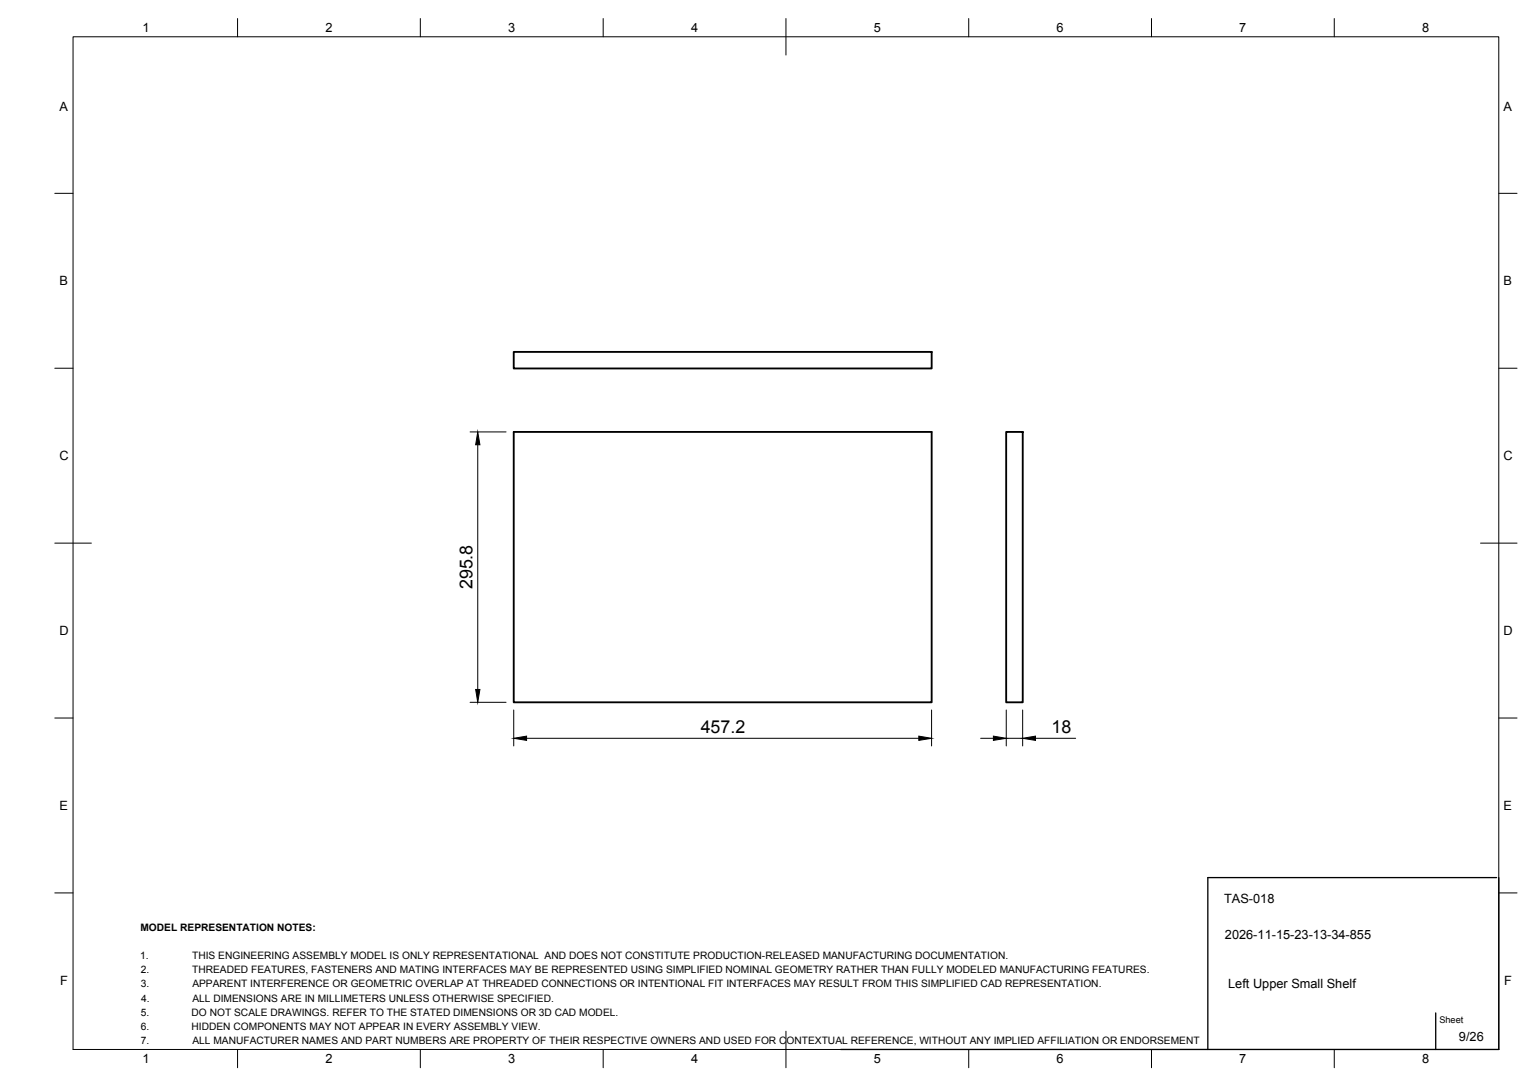
ISO-10303-21;
HEADER;
/* Generated by software containing ST-Developer
 * from STEP Tools, Inc. (www.steptools.com) 
 */

FILE_DESCRIPTION(
/* description */ (''),
/* implementation_level */ '2;1');

FILE_NAME(
/* name */ 'Left Upper Small Shelf.step',
/* time_stamp */ '2026-11-15T15:17:57-08:00',
/* author */ (''),
/* organization */ (''),
/* preprocessor_version */ 'ST-DEVELOPER v20.2',
/* originating_system */ 'Autodesk Translation Framework v15.17.0.0',
/* authorisation */ '');

FILE_SCHEMA (('AUTOMOTIVE_DESIGN { 1 0 10303 214 3 1 1 }'));
ENDSEC;

DATA;
#10=MECHANICAL_DESIGN_GEOMETRIC_PRESENTATION_REPRESENTATION('',(#184),#3723);
#136=SHAPE_REPRESENTATION_RELATIONSHIP('SRR','None',#3817,#160);
#160=ADVANCED_BREP_SHAPE_REPRESENTATION('',(#208),#3706);
#184=STYLED_ITEM('',(#3944),#208);
#208=MANIFOLD_SOLID_BREP('Body1',#2032);
#264=FACE_OUTER_BOUND('',#390,.T.);
#265=FACE_OUTER_BOUND('',#391,.T.);
#266=FACE_OUTER_BOUND('',#392,.T.);
#267=FACE_OUTER_BOUND('',#393,.T.);
#268=FACE_OUTER_BOUND('',#394,.T.);
#269=FACE_OUTER_BOUND('',#395,.T.);
#390=EDGE_LOOP('',(#1461,#1462,#1463,#1464));
#391=EDGE_LOOP('',(#1465,#1466,#1467,#1468));
#392=EDGE_LOOP('',(#1469,#1470,#1471,#1472));
#393=EDGE_LOOP('',(#1473,#1474,#1475,#1476));
#394=EDGE_LOOP('',(#1477,#1478,#1479,#1480));
#395=EDGE_LOOP('',(#1481,#1482,#1483,#1484));
#550=LINE('',#3281,#772);
#551=LINE('',#3283,#773);
#552=LINE('',#3285,#774);
#553=LINE('',#3286,#775);
#554=LINE('',#3289,#776);
#555=LINE('',#3291,#777);
#556=LINE('',#3292,#778);
#557=LINE('',#3295,#779);
#558=LINE('',#3297,#780);
#559=LINE('',#3298,#781);
#560=LINE('',#3300,#782);
#561=LINE('',#3301,#783);
#772=VECTOR('',#2682,0.708661417322828);
#773=VECTOR('',#2683,18.);
#774=VECTOR('',#2684,0.708661417322828);
#775=VECTOR('',#2685,18.);
#776=VECTOR('',#2688,11.6456692913386);
#777=VECTOR('',#2689,11.6456692913386);
#778=VECTOR('',#2690,18.);
#779=VECTOR('',#2693,0.708661417322839);
#780=VECTOR('',#2694,0.708661417322839);
#781=VECTOR('',#2695,18.);
#782=VECTOR('',#2698,11.6456692913386);
#783=VECTOR('',#2699,11.6456692913386);
#971=VERTEX_POINT('',#3279);
#972=VERTEX_POINT('',#3280);
#973=VERTEX_POINT('',#3282);
#974=VERTEX_POINT('',#3284);
#975=VERTEX_POINT('',#3288);
#976=VERTEX_POINT('',#3290);
#977=VERTEX_POINT('',#3294);
#978=VERTEX_POINT('',#3296);
#1152=EDGE_CURVE('',#971,#972,#550,.T.);
#1153=EDGE_CURVE('',#971,#973,#551,.T.);
#1154=EDGE_CURVE('',#973,#974,#552,.T.);
#1155=EDGE_CURVE('',#972,#974,#553,.T.);
#1156=EDGE_CURVE('',#972,#975,#554,.T.);
#1157=EDGE_CURVE('',#974,#976,#555,.T.);
#1158=EDGE_CURVE('',#975,#976,#556,.T.);
#1159=EDGE_CURVE('',#975,#977,#557,.T.);
#1160=EDGE_CURVE('',#976,#978,#558,.T.);
#1161=EDGE_CURVE('',#977,#978,#559,.T.);
#1162=EDGE_CURVE('',#977,#971,#560,.T.);
#1163=EDGE_CURVE('',#978,#973,#561,.T.);
#1461=ORIENTED_EDGE('',*,*,#1152,.F.);
#1462=ORIENTED_EDGE('',*,*,#1153,.T.);
#1463=ORIENTED_EDGE('',*,*,#1154,.T.);
#1464=ORIENTED_EDGE('',*,*,#1155,.F.);
#1465=ORIENTED_EDGE('',*,*,#1156,.F.);
#1466=ORIENTED_EDGE('',*,*,#1155,.T.);
#1467=ORIENTED_EDGE('',*,*,#1157,.T.);
#1468=ORIENTED_EDGE('',*,*,#1158,.F.);
#1469=ORIENTED_EDGE('',*,*,#1159,.F.);
#1470=ORIENTED_EDGE('',*,*,#1158,.T.);
#1471=ORIENTED_EDGE('',*,*,#1160,.T.);
#1472=ORIENTED_EDGE('',*,*,#1161,.F.);
#1473=ORIENTED_EDGE('',*,*,#1162,.F.);
#1474=ORIENTED_EDGE('',*,*,#1161,.T.);
#1475=ORIENTED_EDGE('',*,*,#1163,.T.);
#1476=ORIENTED_EDGE('',*,*,#1153,.F.);
#1477=ORIENTED_EDGE('',*,*,#1154,.F.);
#1478=ORIENTED_EDGE('',*,*,#1163,.F.);
#1479=ORIENTED_EDGE('',*,*,#1160,.F.);
#1480=ORIENTED_EDGE('',*,*,#1157,.F.);
#1481=ORIENTED_EDGE('',*,*,#1162,.T.);
#1482=ORIENTED_EDGE('',*,*,#1152,.T.);
#1483=ORIENTED_EDGE('',*,*,#1156,.T.);
#1484=ORIENTED_EDGE('',*,*,#1159,.T.);
#1817=PLANE('',#2366);
#1818=PLANE('',#2367);
#1819=PLANE('',#2368);
#1820=PLANE('',#2369);
#1821=PLANE('',#2370);
#1822=PLANE('',#2371);
#1938=ADVANCED_FACE('',(#264),#1817,.F.);
#1939=ADVANCED_FACE('',(#265),#1818,.F.);
#1940=ADVANCED_FACE('',(#266),#1819,.F.);
#1941=ADVANCED_FACE('',(#267),#1820,.F.);
#1942=ADVANCED_FACE('',(#268),#1821,.F.);
#1943=ADVANCED_FACE('',(#269),#1822,.T.);
#2032=CLOSED_SHELL('',(#1938,#1939,#1940,#1941,#1942,#1943));
#2365=AXIS2_PLACEMENT_3D('',#3277,#2678,#2679);
#2366=AXIS2_PLACEMENT_3D('',#3278,#2680,#2681);
#2367=AXIS2_PLACEMENT_3D('',#3287,#2686,#2687);
#2368=AXIS2_PLACEMENT_3D('',#3293,#2691,#2692);
#2369=AXIS2_PLACEMENT_3D('',#3299,#2696,#2697);
#2370=AXIS2_PLACEMENT_3D('',#3302,#2700,#2701);
#2371=AXIS2_PLACEMENT_3D('',#3303,#2702,#2703);
#2678=DIRECTION('axis',(0.,0.,1.));
#2679=DIRECTION('refdir',(1.,0.,0.));
#2680=DIRECTION('center_axis',(-1.,0.,0.));
#2681=DIRECTION('ref_axis',(0.,0.,1.));
#2682=DIRECTION('',(0.,1.,0.));
#2683=DIRECTION('',(0.,0.,-1.));
#2684=DIRECTION('',(0.,1.,0.));
#2685=DIRECTION('',(0.,0.,-1.));
#2686=DIRECTION('center_axis',(-7.50657893593751E-16,-1.,0.));
#2687=DIRECTION('ref_axis',(0.,0.,-1.));
#2688=DIRECTION('',(-1.,9.60842103800001E-16,0.));
#2689=DIRECTION('',(-1.,9.60842103800001E-16,0.));
#2690=DIRECTION('',(0.,0.,-1.));
#2691=DIRECTION('center_axis',(1.,0.,0.));
#2692=DIRECTION('ref_axis',(0.,0.,-1.));
#2693=DIRECTION('',(0.,-1.,0.));
#2694=DIRECTION('',(0.,-1.,0.));
#2695=DIRECTION('',(0.,0.,-1.));
#2696=DIRECTION('center_axis',(0.,1.,0.));
#2697=DIRECTION('ref_axis',(0.,0.,1.));
#2698=DIRECTION('',(1.,0.,0.));
#2699=DIRECTION('',(1.,0.,0.));
#2700=DIRECTION('center_axis',(0.,0.,1.));
#2701=DIRECTION('ref_axis',(1.,0.,0.));
#2702=DIRECTION('center_axis',(0.,0.,1.));
#2703=DIRECTION('ref_axis',(1.,0.,0.));
#3277=CARTESIAN_POINT('',(0.,0.,0.));
#3278=CARTESIAN_POINT('Origin',(-0.354330708661419,53.1679790026247,30.375872491424));
#3279=CARTESIAN_POINT('',(-0.354330708661418,52.4593175853018,18.7086614173228));
#3280=CARTESIAN_POINT('',(-0.354330708661419,53.1679790026247,18.7086614173228));
#3281=CARTESIAN_POINT('',(-0.354330708661419,52.4593175853018,18.7086614173228));
#3282=CARTESIAN_POINT('',(-0.354330708661419,52.4593175853018,0.708661417322834));
#3283=CARTESIAN_POINT('',(-0.354330708661419,52.4593175853018,18.7086614173228));
#3284=CARTESIAN_POINT('',(-0.354330708661419,53.1679790026247,0.708661417322834));
#3285=CARTESIAN_POINT('',(-0.354330708661419,52.4593175853018,0.708661417322834));
#3286=CARTESIAN_POINT('',(-0.354330708661419,53.1679790026247,18.7086614173228));
#3287=CARTESIAN_POINT('Origin',(-12.,53.1679790026247,30.375872491424));
#3288=CARTESIAN_POINT('',(-12.,53.1679790026247,18.7086614173228));
#3289=CARTESIAN_POINT('',(-0.35433070866142,53.1679790026247,18.7086614173228));
#3290=CARTESIAN_POINT('',(-12.,53.1679790026247,0.708661417322834));
#3291=CARTESIAN_POINT('',(-0.35433070866142,53.1679790026247,0.708661417322834));
#3292=CARTESIAN_POINT('',(-12.,53.1679790026247,18.7086614173228));
#3293=CARTESIAN_POINT('Origin',(-12.,53.1679790026247,30.375872491424));
#3294=CARTESIAN_POINT('',(-12.,52.4593175853018,18.7086614173228));
#3295=CARTESIAN_POINT('',(-12.,53.1679790026247,18.7086614173228));
#3296=CARTESIAN_POINT('',(-12.,52.4593175853018,0.708661417322834));
#3297=CARTESIAN_POINT('',(-12.,53.1679790026247,0.708661417322834));
#3298=CARTESIAN_POINT('',(-12.,52.4593175853018,18.7086614173228));
#3299=CARTESIAN_POINT('Origin',(-12.,52.4593175853018,30.375872491424));
#3300=CARTESIAN_POINT('',(-12.,52.4593175853018,18.7086614173228));
#3301=CARTESIAN_POINT('',(-12.,52.4593175853018,0.708661417322834));
#3302=CARTESIAN_POINT('Origin',(0.,0.,0.708661417322834));
#3303=CARTESIAN_POINT('Origin',(0.,0.,18.7086614173228));
#3679=UNCERTAINTY_MEASURE_WITH_UNIT(LENGTH_MEASURE(0.000393700787401575),
#3725,'DISTANCE_ACCURACY_VALUE',
'Maximum model space distance between geometric entities at asserted c
onnectivities');
#3696=UNCERTAINTY_MEASURE_WITH_UNIT(LENGTH_MEASURE(0.000393700787401575),
#3725,'DISTANCE_ACCURACY_VALUE',
'Maximum model space distance between geometric entities at asserted c
onnectivities');
#3706=(
GEOMETRIC_REPRESENTATION_CONTEXT(3)
GLOBAL_UNCERTAINTY_ASSIGNED_CONTEXT((#3679))
GLOBAL_UNIT_ASSIGNED_CONTEXT((#3725,#3729,#3730))
REPRESENTATION_CONTEXT('','3D')
);
#3723=(
GEOMETRIC_REPRESENTATION_CONTEXT(3)
GLOBAL_UNCERTAINTY_ASSIGNED_CONTEXT((#3696))
GLOBAL_UNIT_ASSIGNED_CONTEXT((#3725,#3729,#3730))
REPRESENTATION_CONTEXT('','3D')
);
#3724=DIMENSIONAL_EXPONENTS(1.,0.,0.,0.,0.,0.,0.);
#3725=(
CONVERSION_BASED_UNIT('inch',#3728)
LENGTH_UNIT()
NAMED_UNIT(#3724)
);
#3726=(
LENGTH_UNIT()
NAMED_UNIT(*)
SI_UNIT(.MILLI.,.METRE.)
);
#3728=LENGTH_MEASURE_WITH_UNIT(LENGTH_MEASURE(25.4),#3726);
#3729=(
NAMED_UNIT(*)
PLANE_ANGLE_UNIT()
SI_UNIT($,.RADIAN.)
);
#3730=(
NAMED_UNIT(*)
SI_UNIT($,.STERADIAN.)
SOLID_ANGLE_UNIT()
);
#3740=SHAPE_DEFINITION_REPRESENTATION(#3767,#3817);
#3767=PRODUCT_DEFINITION_SHAPE('',$,#3844);
#3817=SHAPE_REPRESENTATION('',(#2365),#3706);
#3834=PRODUCT_DEFINITION_CONTEXT('part definition',#3914,'design');
#3844=PRODUCT_DEFINITION('2026-11-15-23-13-34-855',
'Left Upper Small Shelf',#3870,#3834);
#3870=PRODUCT_DEFINITION_FORMATION('',$,#3925);
#3914=APPLICATION_CONTEXT(
'Core Data for Automotive Mechanical Design Process');
#3915=PRODUCT_CONTEXT('part definition',#3914,'mechanical');
#3925=PRODUCT('2026-11-15-23-13-34-855','Left Upper Small Shelf',$,(#3915));
#3944=PRESENTATION_STYLE_ASSIGNMENT((#3952));
#3952=SURFACE_STYLE_USAGE(.BOTH.,#3960);
#3960=SURFACE_SIDE_STYLE('',(#3968));
#3968=SURFACE_STYLE_FILL_AREA(#3976);
#3976=FILL_AREA_STYLE('Light Gray',(#3984));
#3984=FILL_AREA_STYLE_COLOUR('Light Gray',#3992);
#3992=COLOUR_RGB('Light Gray',0.827450980392157,0.827450980392157,0.827450980392157);
ENDSEC;
END-ISO-10303-21;
